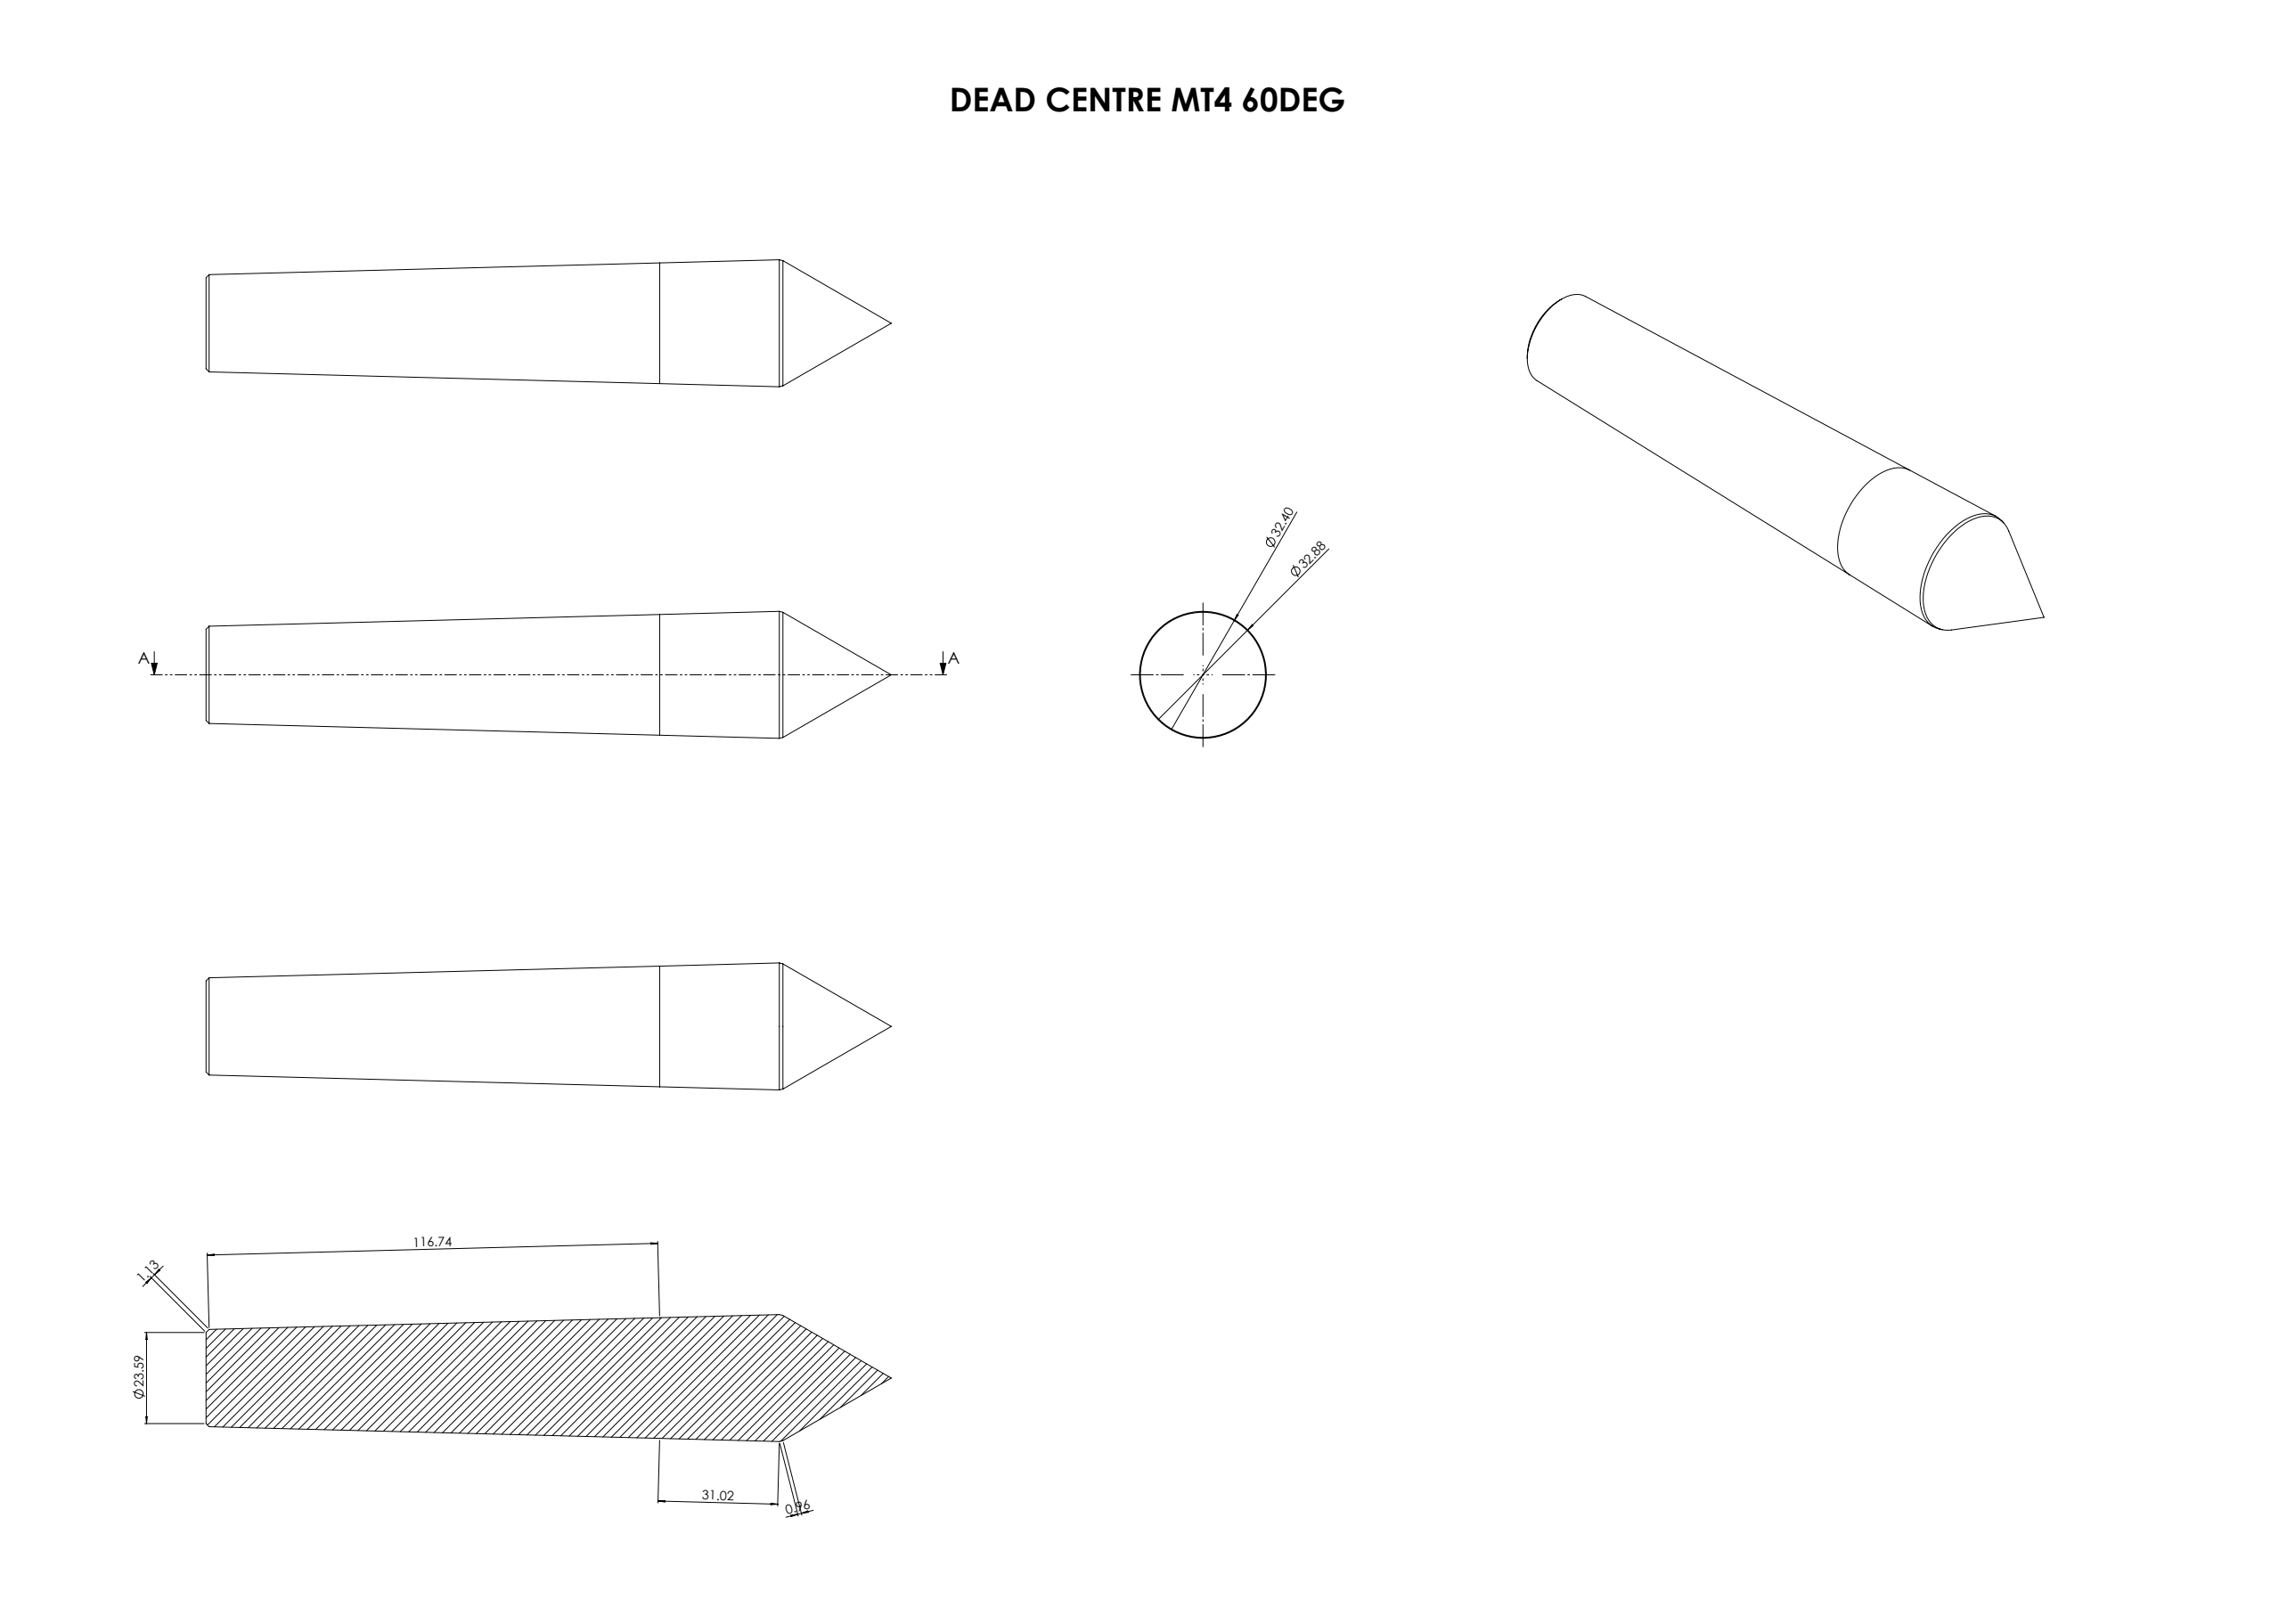
ISO-10303-21;
HEADER;
/* Generated by software containing ST-Developer
 * from STEP Tools, Inc. (www.steptools.com) 
 */

FILE_DESCRIPTION(
/* description */ (''),
/* implementation_level */ '2;1');

FILE_NAME(
/* name */ '04_Dead_Centre_MT4_60deg.step',
/* time_stamp */ '2026-10-26T03:50:32-07:00',
/* author */ (''),
/* organization */ (''),
/* preprocessor_version */ 'ST-DEVELOPER v20.2',
/* originating_system */ 'Autodesk Translation Framework v15.15.0.0',
/* authorisation */ '');

FILE_SCHEMA (('AUTOMOTIVE_DESIGN { 1 0 10303 214 3 1 1 }'));
ENDSEC;

DATA;
#10=MECHANICAL_DESIGN_GEOMETRIC_PRESENTATION_REPRESENTATION('',(#1042),#76660);
#1002=SHAPE_REPRESENTATION_RELATIONSHIP('SRR','None',#76739,#1022);
#1022=ADVANCED_BREP_SHAPE_REPRESENTATION('',(#1062),#76643);
#1042=STYLED_ITEM('',(#76892),#1062);
#1062=MANIFOLD_SOLID_BREP('Dead centre',#26667);
#1916=PLANE('',#27584);
#2955=FACE_OUTER_BOUND('',#4560,.T.);
#2956=FACE_OUTER_BOUND('',#4561,.T.);
#2957=FACE_OUTER_BOUND('',#4562,.T.);
#2958=FACE_OUTER_BOUND('',#4563,.T.);
#2959=FACE_OUTER_BOUND('',#4564,.T.);
#2960=FACE_OUTER_BOUND('',#4565,.T.);
#4560=EDGE_LOOP('',(#19221,#19222,#19223,#19224,#19225,#19226));
#4561=EDGE_LOOP('',(#19227,#19228,#19229,#19230,#19231));
#4562=EDGE_LOOP('',(#19232,#19233,#19234,#19235));
#4563=EDGE_LOOP('',(#19236));
#4564=EDGE_LOOP('',(#19237,#19238,#19239,#19240));
#4565=EDGE_LOOP('',(#19241,#19242,#19243,#19244));
#5976=CIRCLE('',#27577,1.62016810220205);
#5977=CIRCLE('',#27578,1.62016810220205);
#5978=CIRCLE('',#27579,1.64385418552926);
#5979=CIRCLE('',#27580,1.64385418552926);
#5980=CIRCLE('',#27582,1.56235);
#5981=CIRCLE('',#27585,1.1792801);
#5982=CIRCLE('',#27587,1.2592801);
#7290=LINE('',#40074,#9446);
#7291=LINE('',#40080,#9447);
#7292=LINE('',#40084,#9448);
#7293=LINE('',#40091,#9449);
#7294=LINE('',#40093,#9450);
#9446=VECTOR('',#31391,1.63201114386566);
#9447=VECTOR('',#31398,1.60375905110103);
#9448=VECTOR('',#31403,1.64516810220205);
#9449=VECTOR('',#31412,1.2192801);
#9450=VECTOR('',#31415,1.41081505);
#11526=VERTEX_POINT('',#40069);
#11527=VERTEX_POINT('',#40070);
#11528=VERTEX_POINT('',#40073);
#11529=VERTEX_POINT('',#40075);
#11530=VERTEX_POINT('',#40079);
#11531=VERTEX_POINT('',#40083);
#11532=VERTEX_POINT('',#40086);
#11533=VERTEX_POINT('',#40089);
#14333=EDGE_CURVE('',#11526,#11527,#5976,.T.);
#14334=EDGE_CURVE('',#11527,#11526,#5977,.T.);
#14335=EDGE_CURVE('',#11526,#11528,#7290,.T.);
#14336=EDGE_CURVE('',#11528,#11529,#5978,.T.);
#14337=EDGE_CURVE('',#11529,#11528,#5979,.T.);
#14338=EDGE_CURVE('',#11529,#11530,#7291,.T.);
#14339=EDGE_CURVE('',#11530,#11530,#5980,.T.);
#14340=EDGE_CURVE('',#11531,#11527,#7292,.T.);
#14341=EDGE_CURVE('',#11532,#11532,#5981,.T.);
#14342=EDGE_CURVE('',#11533,#11533,#5982,.T.);
#14343=EDGE_CURVE('',#11533,#11532,#7293,.T.);
#14344=EDGE_CURVE('',#11530,#11533,#7294,.T.);
#19221=ORIENTED_EDGE('',*,*,#14333,.T.);
#19222=ORIENTED_EDGE('',*,*,#14334,.T.);
#19223=ORIENTED_EDGE('',*,*,#14335,.T.);
#19224=ORIENTED_EDGE('',*,*,#14336,.T.);
#19225=ORIENTED_EDGE('',*,*,#14337,.T.);
#19226=ORIENTED_EDGE('',*,*,#14335,.F.);
#19227=ORIENTED_EDGE('',*,*,#14336,.F.);
#19228=ORIENTED_EDGE('',*,*,#14337,.F.);
#19229=ORIENTED_EDGE('',*,*,#14338,.T.);
#19230=ORIENTED_EDGE('',*,*,#14339,.T.);
#19231=ORIENTED_EDGE('',*,*,#14338,.F.);
#19232=ORIENTED_EDGE('',*,*,#14340,.T.);
#19233=ORIENTED_EDGE('',*,*,#14333,.F.);
#19234=ORIENTED_EDGE('',*,*,#14334,.F.);
#19235=ORIENTED_EDGE('',*,*,#14340,.F.);
#19236=ORIENTED_EDGE('',*,*,#14341,.F.);
#19237=ORIENTED_EDGE('',*,*,#14342,.F.);
#19238=ORIENTED_EDGE('',*,*,#14343,.T.);
#19239=ORIENTED_EDGE('',*,*,#14341,.T.);
#19240=ORIENTED_EDGE('',*,*,#14343,.F.);
#19241=ORIENTED_EDGE('',*,*,#14339,.F.);
#19242=ORIENTED_EDGE('',*,*,#14344,.T.);
#19243=ORIENTED_EDGE('',*,*,#14342,.T.);
#19244=ORIENTED_EDGE('',*,*,#14344,.F.);
#25013=CONICAL_SURFACE('',#27576,1.63201114386566,0.248658708390703);
#25014=CONICAL_SURFACE('',#27581,1.60375905110103,0.0262813588168537);
#25015=CONICAL_SURFACE('',#27583,1.64516810220205,0.523598775598299);
#25016=CONICAL_SURFACE('',#27586,1.2192801,0.785398163397437);
#25017=CONICAL_SURFACE('',#27588,1.41081505,0.0259641639514023);
#25543=ADVANCED_FACE('',(#2955),#25013,.T.);
#25544=ADVANCED_FACE('',(#2956),#25014,.T.);
#25545=ADVANCED_FACE('',(#2957),#25015,.T.);
#25546=ADVANCED_FACE('',(#2958),#1916,.T.);
#25547=ADVANCED_FACE('',(#2959),#25016,.T.);
#25548=ADVANCED_FACE('',(#2960),#25017,.T.);
#26667=CLOSED_SHELL('',(#25543,#25544,#25545,#25546,#25547,#25548));
#27575=AXIS2_PLACEMENT_3D('',#40067,#31383,#31384);
#27576=AXIS2_PLACEMENT_3D('',#40068,#31385,#31386);
#27577=AXIS2_PLACEMENT_3D('',#40071,#31387,#31388);
#27578=AXIS2_PLACEMENT_3D('',#40072,#31389,#31390);
#27579=AXIS2_PLACEMENT_3D('',#40076,#31392,#31393);
#27580=AXIS2_PLACEMENT_3D('',#40077,#31394,#31395);
#27581=AXIS2_PLACEMENT_3D('',#40078,#31396,#31397);
#27582=AXIS2_PLACEMENT_3D('',#40081,#31399,#31400);
#27583=AXIS2_PLACEMENT_3D('',#40082,#31401,#31402);
#27584=AXIS2_PLACEMENT_3D('',#40085,#31404,#31405);
#27585=AXIS2_PLACEMENT_3D('',#40087,#31406,#31407);
#27586=AXIS2_PLACEMENT_3D('',#40088,#31408,#31409);
#27587=AXIS2_PLACEMENT_3D('',#40090,#31410,#31411);
#27588=AXIS2_PLACEMENT_3D('',#40092,#31413,#31414);
#31383=DIRECTION('axis',(0.,0.,1.));
#31384=DIRECTION('refdir',(1.,0.,0.));
#31385=DIRECTION('center_axis',(-1.,0.,0.));
#31386=DIRECTION('ref_axis',(0.,-1.,0.));
#31387=DIRECTION('center_axis',(-1.,0.,0.));
#31388=DIRECTION('ref_axis',(0.,-1.,0.));
#31389=DIRECTION('center_axis',(-1.,0.,0.));
#31390=DIRECTION('ref_axis',(0.,-1.,0.));
#31391=DIRECTION('',(-0.969243390898598,0.246104142995171,3.01390650975938E-17));
#31392=DIRECTION('center_axis',(1.,0.,0.));
#31393=DIRECTION('ref_axis',(0.,-1.,0.));
#31394=DIRECTION('center_axis',(1.,0.,0.));
#31395=DIRECTION('ref_axis',(0.,-1.,0.));
#31396=DIRECTION('center_axis',(1.,0.,0.));
#31397=DIRECTION('ref_axis',(0.,1.,0.));
#31398=DIRECTION('',(-0.999654664967248,0.0262783334558961,3.218167695369E-18));
#31399=DIRECTION('center_axis',(1.,0.,0.));
#31400=DIRECTION('ref_axis',(0.,0.,-1.));
#31401=DIRECTION('center_axis',(-1.,0.,0.));
#31402=DIRECTION('ref_axis',(0.,1.,0.));
#31403=DIRECTION('',(-0.866025403784439,-0.5,-6.12323399573677E-17));
#31404=DIRECTION('center_axis',(-1.,0.,0.));
#31405=DIRECTION('ref_axis',(0.,0.,1.));
#31406=DIRECTION('center_axis',(1.,0.,0.));
#31407=DIRECTION('ref_axis',(0.,0.,-1.));
#31408=DIRECTION('center_axis',(1.,0.,0.));
#31409=DIRECTION('ref_axis',(0.,1.,0.));
#31410=DIRECTION('center_axis',(1.,0.,0.));
#31411=DIRECTION('ref_axis',(0.,0.,-1.));
#31412=DIRECTION('',(-0.707106781186555,0.70710678118654,8.65956056235484E-17));
#31413=DIRECTION('center_axis',(1.,0.,0.));
#31414=DIRECTION('ref_axis',(0.,1.,0.));
#31415=DIRECTION('',(-0.999662950030635,0.0259612468122956,3.17933578105522E-18));
#40067=CARTESIAN_POINT('',(0.,0.,0.));
#40068=CARTESIAN_POINT('Origin',(42.1471445284648,0.,26.5));
#40069=CARTESIAN_POINT('',(42.1937865301836,1.62016810220205,26.5));
#40070=CARTESIAN_POINT('',(42.1937865301836,-1.62016810220206,26.5));
#40071=CARTESIAN_POINT('Origin',(42.1937865301836,0.,26.5));
#40072=CARTESIAN_POINT('Origin',(42.1937865301836,0.,26.5));
#40073=CARTESIAN_POINT('',(42.100502526746,1.64385418552926,26.5));
#40074=CARTESIAN_POINT('',(42.1471445284648,1.63201114386566,26.5));
#40075=CARTESIAN_POINT('',(42.100502526746,-1.64385418552926,26.5));
#40076=CARTESIAN_POINT('Origin',(42.100502526746,0.,26.5));
#40077=CARTESIAN_POINT('Origin',(42.100502526746,0.,26.5));
#40078=CARTESIAN_POINT('Origin',(40.5752426299972,0.,26.5));
#40079=CARTESIAN_POINT('',(39.,-1.56235,26.5));
#40080=CARTESIAN_POINT('',(40.5752426299972,-1.60375905110103,26.5));
#40081=CARTESIAN_POINT('Origin',(39.,0.,26.5));
#40082=CARTESIAN_POINT('Origin',(42.1504852599944,0.,26.5));
#40083=CARTESIAN_POINT('',(45.,0.,26.5));
#40084=CARTESIAN_POINT('',(42.1504852599944,-1.64516810220205,26.5));
#40085=CARTESIAN_POINT('Origin',(27.25,1.1792801,26.5));
#40086=CARTESIAN_POINT('',(27.25,-1.1792801,26.5));
#40087=CARTESIAN_POINT('Origin',(27.25,0.,26.5));
#40088=CARTESIAN_POINT('Origin',(27.29,0.,26.5));
#40089=CARTESIAN_POINT('',(27.33,-1.2592801,26.5));
#40090=CARTESIAN_POINT('Origin',(27.33,0.,26.5));
#40091=CARTESIAN_POINT('',(27.29,-1.2192801,26.5));
#40092=CARTESIAN_POINT('Origin',(33.165,0.,26.5));
#40093=CARTESIAN_POINT('',(33.165,-1.41081505,26.5));
#76621=UNCERTAINTY_MEASURE_WITH_UNIT(LENGTH_MEASURE(0.001),#76661,
'DISTANCE_ACCURACY_VALUE',
'Maximum model space distance between geometric entities at asserted c
onnectivities');
#76638=UNCERTAINTY_MEASURE_WITH_UNIT(LENGTH_MEASURE(0.001),#76661,
'DISTANCE_ACCURACY_VALUE',
'Maximum model space distance between geometric entities at asserted c
onnectivities');
#76643=(
GEOMETRIC_REPRESENTATION_CONTEXT(3)
GLOBAL_UNCERTAINTY_ASSIGNED_CONTEXT((#76621))
GLOBAL_UNIT_ASSIGNED_CONTEXT((#76661,#76663,#76664))
REPRESENTATION_CONTEXT('','3D')
);
#76660=(
GEOMETRIC_REPRESENTATION_CONTEXT(3)
GLOBAL_UNCERTAINTY_ASSIGNED_CONTEXT((#76638))
GLOBAL_UNIT_ASSIGNED_CONTEXT((#76661,#76663,#76664))
REPRESENTATION_CONTEXT('','3D')
);
#76661=(
LENGTH_UNIT()
NAMED_UNIT(*)
SI_UNIT(.CENTI.,.METRE.)
);
#76663=(
NAMED_UNIT(*)
PLANE_ANGLE_UNIT()
SI_UNIT($,.RADIAN.)
);
#76664=(
NAMED_UNIT(*)
SI_UNIT($,.STERADIAN.)
SOLID_ANGLE_UNIT()
);
#76669=SHAPE_DEFINITION_REPRESENTATION(#76690,#76739);
#76690=PRODUCT_DEFINITION_SHAPE('',$,#76761);
#76739=SHAPE_REPRESENTATION('',(#27575),#76643);
#76756=PRODUCT_DEFINITION_CONTEXT('part definition',#76821,'design');
#76761=PRODUCT_DEFINITION('2026-10-26-11-12-44-090',
'04_Dead_Centre_MT4_60deg',#76782,#76756);
#76782=PRODUCT_DEFINITION_FORMATION('',$,#76827);
#76821=APPLICATION_CONTEXT(
'Core Data for Automotive Mechanical Design Process');
#76822=PRODUCT_CONTEXT('part definition',#76821,'mechanical');
#76827=PRODUCT('2026-10-26-11-12-44-090','04_Dead_Centre_MT4_60deg',$,(#76822));
#76886=COLOUR_RGB('Light Blue',0.38,0.62,0.78);
#76887=FILL_AREA_STYLE_COLOUR('',#76886);
#76888=FILL_AREA_STYLE('',(#76887));
#76889=SURFACE_STYLE_FILL_AREA(#76888);
#76890=SURFACE_SIDE_STYLE('',(#76889));
#76891=SURFACE_STYLE_USAGE(.BOTH.,#76890);
#76892=PRESENTATION_STYLE_ASSIGNMENT((#76891));
ENDSEC;
END-ISO-10303-21;
